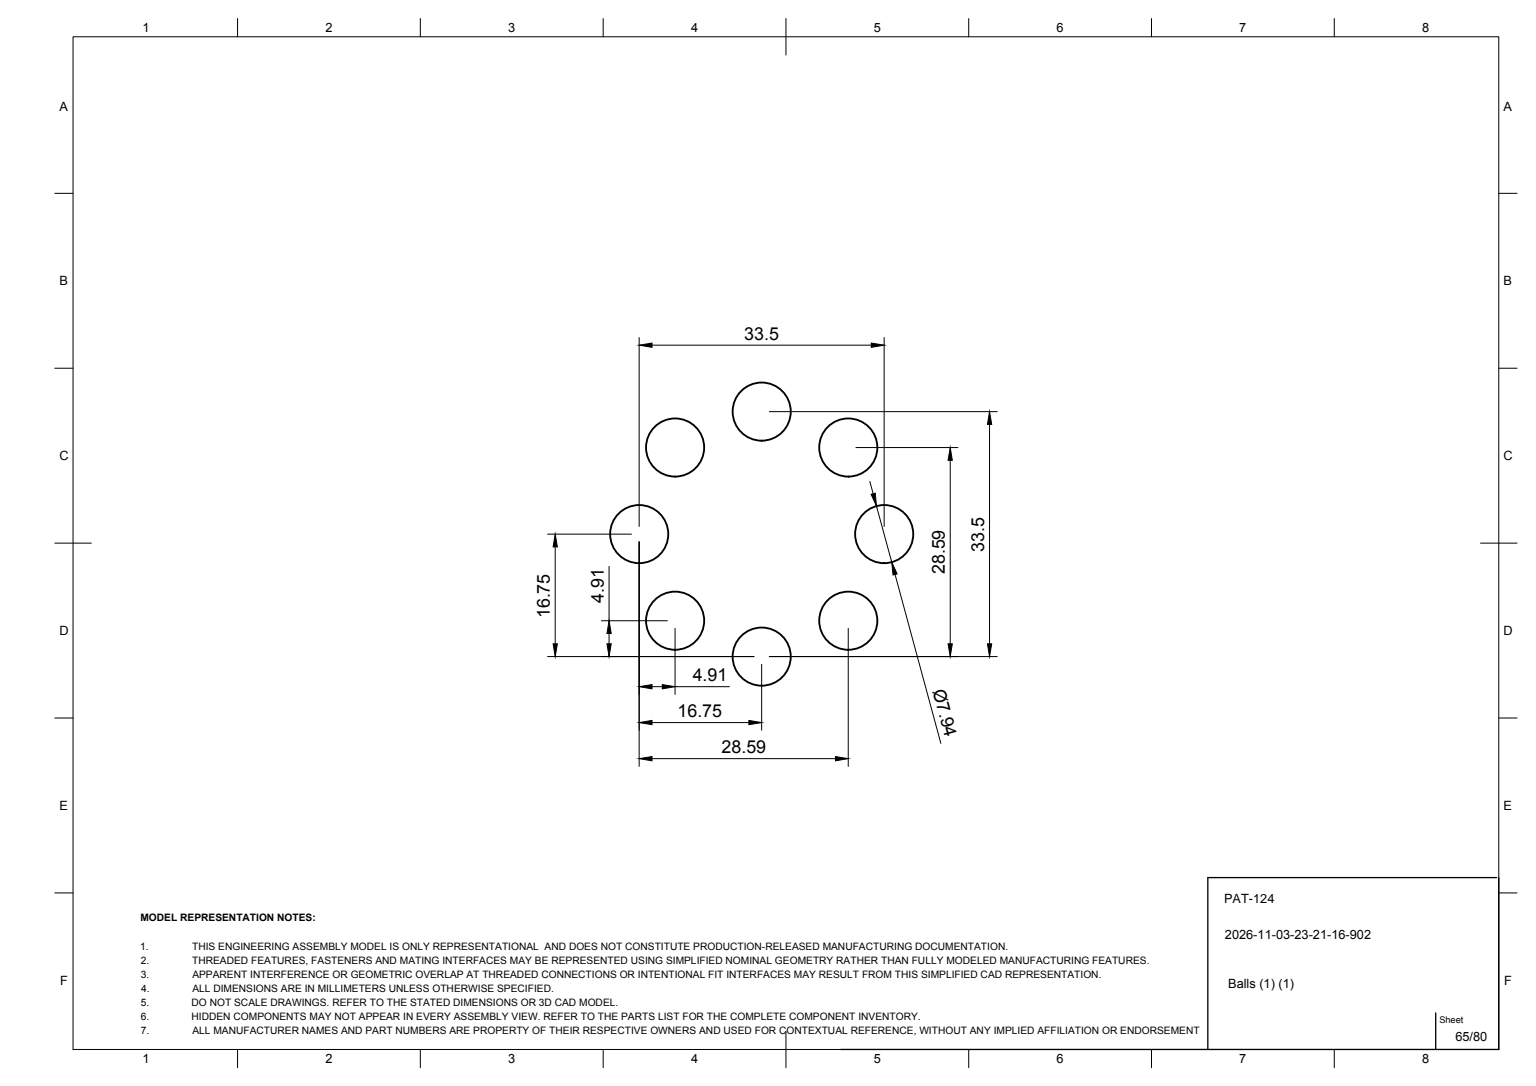
ISO-10303-21;
HEADER;
/* Generated by software containing ST-Developer
 * from STEP Tools, Inc. (www.steptools.com) 
 */

FILE_DESCRIPTION(
/* description */ ('XY cross-slide table'),
/* implementation_level */ '2;1');

FILE_NAME(
/* name */ 'Balls (1) (1).step',
/* time_stamp */ '2026-10-28T03:22:46-07:00',
/* author */ (''),
/* organization */ (''),
/* preprocessor_version */ 'ST-DEVELOPER v20.2',
/* originating_system */ 'Autodesk Translation Framework v15.17.0.0',
/* authorisation */ '');

FILE_SCHEMA (('AUTOMOTIVE_DESIGN { 1 0 10303 214 3 1 1 }'));
ENDSEC;

DATA;
#10=MECHANICAL_DESIGN_GEOMETRIC_PRESENTATION_REPRESENTATION('',(#1750,#1751,#1752,#1753,#1754,#1755,#1756,#1757),#62984);
#1425=SPHERICAL_SURFACE('',#25700,0.3969);
#1426=SPHERICAL_SURFACE('',#25702,0.3969);
#1427=SPHERICAL_SURFACE('',#25704,0.3969);
#1428=SPHERICAL_SURFACE('',#25706,0.3969);
#1429=SPHERICAL_SURFACE('',#25708,0.3969);
#1430=SPHERICAL_SURFACE('',#25710,0.3969);
#1431=SPHERICAL_SURFACE('',#25712,0.3969);
#1432=SPHERICAL_SURFACE('',#25714,0.3969);
#1562=SHAPE_REPRESENTATION_RELATIONSHIP('SRR','None',#63419,#1645);
#1645=ADVANCED_BREP_SHAPE_REPRESENTATION('',(#1859,#1860,#1861,#1862,#1863,
#1864,#1865,#1866),#62956);
#1750=STYLED_ITEM('',(#63905),#1859);
#1751=STYLED_ITEM('',(#63905),#1860);
#1752=STYLED_ITEM('',(#63905),#1861);
#1753=STYLED_ITEM('',(#63905),#1862);
#1754=STYLED_ITEM('',(#63905),#1863);
#1755=STYLED_ITEM('',(#63905),#1864);
#1756=STYLED_ITEM('',(#63905),#1865);
#1757=STYLED_ITEM('',(#63905),#1866);
#1859=MANIFOLD_SOLID_BREP('Body1',#23048);
#1860=MANIFOLD_SOLID_BREP('Body2',#23049);
#1861=MANIFOLD_SOLID_BREP('Body3',#23050);
#1862=MANIFOLD_SOLID_BREP('Body4',#23051);
#1863=MANIFOLD_SOLID_BREP('Body5',#23052);
#1864=MANIFOLD_SOLID_BREP('Body6',#23053);
#1865=MANIFOLD_SOLID_BREP('Body7',#23054);
#1866=MANIFOLD_SOLID_BREP('Body8',#23055);
#3739=FACE_OUTER_BOUND('',#5380,.T.);
#3740=FACE_OUTER_BOUND('',#5381,.T.);
#3741=FACE_OUTER_BOUND('',#5382,.T.);
#3742=FACE_OUTER_BOUND('',#5383,.T.);
#3743=FACE_OUTER_BOUND('',#5384,.T.);
#3744=FACE_OUTER_BOUND('',#5385,.T.);
#3745=FACE_OUTER_BOUND('',#5386,.T.);
#3746=FACE_OUTER_BOUND('',#5387,.T.);
#5380=EDGE_LOOP('',(#18890,#18891));
#5381=EDGE_LOOP('',(#18892,#18893));
#5382=EDGE_LOOP('',(#18894,#18895));
#5383=EDGE_LOOP('',(#18896,#18897));
#5384=EDGE_LOOP('',(#18898,#18899));
#5385=EDGE_LOOP('',(#18900,#18901));
#5386=EDGE_LOOP('',(#18902,#18903));
#5387=EDGE_LOOP('',(#18904,#18905));
#9558=CIRCLE('',#25701,0.3969);
#9559=CIRCLE('',#25703,0.3969);
#9560=CIRCLE('',#25705,0.3969);
#9561=CIRCLE('',#25707,0.3969);
#9562=CIRCLE('',#25709,0.3969);
#9563=CIRCLE('',#25711,0.3969);
#9564=CIRCLE('',#25713,0.3969);
#9565=CIRCLE('',#25715,0.3969);
#11115=VERTEX_POINT('',#49131);
#11116=VERTEX_POINT('',#49132);
#11117=VERTEX_POINT('',#49135);
#11118=VERTEX_POINT('',#49136);
#11119=VERTEX_POINT('',#49139);
#11120=VERTEX_POINT('',#49140);
#11121=VERTEX_POINT('',#49143);
#11122=VERTEX_POINT('',#49144);
#11123=VERTEX_POINT('',#49147);
#11124=VERTEX_POINT('',#49148);
#11125=VERTEX_POINT('',#49151);
#11126=VERTEX_POINT('',#49152);
#11127=VERTEX_POINT('',#49155);
#11128=VERTEX_POINT('',#49156);
#11129=VERTEX_POINT('',#49159);
#11130=VERTEX_POINT('',#49160);
#13829=EDGE_CURVE('',#11115,#11116,#9558,.T.);
#13830=EDGE_CURVE('',#11117,#11118,#9559,.T.);
#13831=EDGE_CURVE('',#11119,#11120,#9560,.T.);
#13832=EDGE_CURVE('',#11121,#11122,#9561,.T.);
#13833=EDGE_CURVE('',#11123,#11124,#9562,.T.);
#13834=EDGE_CURVE('',#11125,#11126,#9563,.T.);
#13835=EDGE_CURVE('',#11127,#11128,#9564,.T.);
#13836=EDGE_CURVE('',#11129,#11130,#9565,.T.);
#18890=ORIENTED_EDGE('',*,*,#13829,.T.);
#18891=ORIENTED_EDGE('',*,*,#13829,.F.);
#18892=ORIENTED_EDGE('',*,*,#13830,.T.);
#18893=ORIENTED_EDGE('',*,*,#13830,.F.);
#18894=ORIENTED_EDGE('',*,*,#13831,.T.);
#18895=ORIENTED_EDGE('',*,*,#13831,.F.);
#18896=ORIENTED_EDGE('',*,*,#13832,.T.);
#18897=ORIENTED_EDGE('',*,*,#13832,.F.);
#18898=ORIENTED_EDGE('',*,*,#13833,.T.);
#18899=ORIENTED_EDGE('',*,*,#13833,.F.);
#18900=ORIENTED_EDGE('',*,*,#13834,.T.);
#18901=ORIENTED_EDGE('',*,*,#13834,.F.);
#18902=ORIENTED_EDGE('',*,*,#13835,.T.);
#18903=ORIENTED_EDGE('',*,*,#13835,.F.);
#18904=ORIENTED_EDGE('',*,*,#13836,.T.);
#18905=ORIENTED_EDGE('',*,*,#13836,.F.);
#22520=ADVANCED_FACE('',(#3739),#1425,.T.);
#22521=ADVANCED_FACE('',(#3740),#1426,.T.);
#22522=ADVANCED_FACE('',(#3741),#1427,.T.);
#22523=ADVANCED_FACE('',(#3742),#1428,.T.);
#22524=ADVANCED_FACE('',(#3743),#1429,.T.);
#22525=ADVANCED_FACE('',(#3744),#1430,.T.);
#22526=ADVANCED_FACE('',(#3745),#1431,.T.);
#22527=ADVANCED_FACE('',(#3746),#1432,.T.);
#23048=CLOSED_SHELL('',(#22520));
#23049=CLOSED_SHELL('',(#22521));
#23050=CLOSED_SHELL('',(#22522));
#23051=CLOSED_SHELL('',(#22523));
#23052=CLOSED_SHELL('',(#22524));
#23053=CLOSED_SHELL('',(#22525));
#23054=CLOSED_SHELL('',(#22526));
#23055=CLOSED_SHELL('',(#22527));
#25699=AXIS2_PLACEMENT_3D('',#49129,#30816,#30817);
#25700=AXIS2_PLACEMENT_3D('',#49130,#30818,#30819);
#25701=AXIS2_PLACEMENT_3D('',#49133,#30820,#30821);
#25702=AXIS2_PLACEMENT_3D('',#49134,#30822,#30823);
#25703=AXIS2_PLACEMENT_3D('',#49137,#30824,#30825);
#25704=AXIS2_PLACEMENT_3D('',#49138,#30826,#30827);
#25705=AXIS2_PLACEMENT_3D('',#49141,#30828,#30829);
#25706=AXIS2_PLACEMENT_3D('',#49142,#30830,#30831);
#25707=AXIS2_PLACEMENT_3D('',#49145,#30832,#30833);
#25708=AXIS2_PLACEMENT_3D('',#49146,#30834,#30835);
#25709=AXIS2_PLACEMENT_3D('',#49149,#30836,#30837);
#25710=AXIS2_PLACEMENT_3D('',#49150,#30838,#30839);
#25711=AXIS2_PLACEMENT_3D('',#49153,#30840,#30841);
#25712=AXIS2_PLACEMENT_3D('',#49154,#30842,#30843);
#25713=AXIS2_PLACEMENT_3D('',#49157,#30844,#30845);
#25714=AXIS2_PLACEMENT_3D('',#49158,#30846,#30847);
#25715=AXIS2_PLACEMENT_3D('',#49161,#30848,#30849);
#30816=DIRECTION('axis',(0.,0.,1.));
#30817=DIRECTION('refdir',(1.,0.,0.));
#30818=DIRECTION('center_axis',(0.,0.,1.));
#30819=DIRECTION('ref_axis',(1.,0.,0.));
#30820=DIRECTION('center_axis',(1.22464679914735E-16,-1.,0.));
#30821=DIRECTION('ref_axis',(-1.,-1.22464679914735E-16,0.));
#30822=DIRECTION('center_axis',(0.707106781186548,0.,0.707106781186548));
#30823=DIRECTION('ref_axis',(0.707106781186548,0.,-0.707106781186548));
#30824=DIRECTION('center_axis',(8.65956056235493E-17,-1.,-8.65956056235493E-17));
#30825=DIRECTION('ref_axis',(-0.707106781186548,-1.22464679914735E-16,0.707106781186548));
#30826=DIRECTION('center_axis',(1.,0.,0.));
#30827=DIRECTION('ref_axis',(6.12323399573677E-17,0.,-1.));
#30828=DIRECTION('center_axis',(7.49879891330929E-33,-1.,-1.22464679914735E-16));
#30829=DIRECTION('ref_axis',(-6.12323399573677E-17,-1.22464679914735E-16,
1.));
#30830=DIRECTION('center_axis',(0.707106781186548,0.,-0.707106781186548));
#30831=DIRECTION('ref_axis',(-0.707106781186548,0.,-0.707106781186548));
#30832=DIRECTION('center_axis',(-8.65956056235493E-17,-1.,-8.65956056235493E-17));
#30833=DIRECTION('ref_axis',(0.707106781186548,-1.22464679914735E-16,0.707106781186548));
#30834=DIRECTION('center_axis',(0.,0.,-1.));
#30835=DIRECTION('ref_axis',(-1.,0.,-1.22464679914735E-16));
#30836=DIRECTION('center_axis',(-1.22464679914735E-16,-1.,-1.49975978266186E-32));
#30837=DIRECTION('ref_axis',(1.,-1.22464679914735E-16,1.22464679914735E-16));
#30838=DIRECTION('center_axis',(-0.707106781186548,0.,-0.707106781186548));
#30839=DIRECTION('ref_axis',(-0.707106781186548,0.,0.707106781186548));
#30840=DIRECTION('center_axis',(-8.65956056235493E-17,-1.,8.65956056235493E-17));
#30841=DIRECTION('ref_axis',(0.707106781186548,-1.22464679914735E-16,-0.707106781186548));
#30842=DIRECTION('center_axis',(-1.,0.,0.));
#30843=DIRECTION('ref_axis',(-1.83697019872103E-16,0.,1.));
#30844=DIRECTION('center_axis',(-2.24963967399279E-32,-1.,1.22464679914735E-16));
#30845=DIRECTION('ref_axis',(1.83697019872103E-16,-1.22464679914735E-16,
-1.));
#30846=DIRECTION('center_axis',(-0.707106781186548,0.,0.707106781186548));
#30847=DIRECTION('ref_axis',(0.707106781186548,0.,0.707106781186548));
#30848=DIRECTION('center_axis',(8.65956056235493E-17,-1.,8.65956056235494E-17));
#30849=DIRECTION('ref_axis',(-0.707106781186548,-1.22464679914735E-16,-0.707106781186548));
#49129=CARTESIAN_POINT('',(0.,0.,0.));
#49130=CARTESIAN_POINT('Origin',(1.675,0.,0.));
#49131=CARTESIAN_POINT('',(1.675,-2.97627328869245E-33,0.3969));
#49132=CARTESIAN_POINT('',(1.675,-2.97627328869245E-33,-0.3969));
#49133=CARTESIAN_POINT('Origin',(1.675,0.,0.));
#49134=CARTESIAN_POINT('Origin',(1.18440385848747,0.,-1.18440385848747));
#49135=CARTESIAN_POINT('',(1.46505453994041,3.1867025333467E-33,-0.903753177034526));
#49136=CARTESIAN_POINT('',(0.903753177034527,-9.13924911073161E-33,-1.46505453994041));
#49137=CARTESIAN_POINT('Origin',(1.18440385848747,0.,-1.18440385848747));
#49138=CARTESIAN_POINT('Origin',(1.02564169428591E-16,0.,-1.675));
#49139=CARTESIAN_POINT('',(0.3969,-2.97627328869246E-33,-1.675));
#49140=CARTESIAN_POINT('',(-0.3969,-2.97627328869245E-33,-1.675));
#49141=CARTESIAN_POINT('Origin',(1.02564169428591E-16,0.,-1.675));
#49142=CARTESIAN_POINT('Origin',(-1.18440385848747,0.,-1.18440385848747));
#49143=CARTESIAN_POINT('',(-0.903753177034526,3.1867025333467E-33,-1.46505453994041));
#49144=CARTESIAN_POINT('',(-1.46505453994041,-9.13924911073161E-33,-0.903753177034527));
#49145=CARTESIAN_POINT('Origin',(-1.18440385848747,0.,-1.18440385848747));
#49146=CARTESIAN_POINT('Origin',(-1.675,0.,-2.05128338857182E-16));
#49147=CARTESIAN_POINT('',(-1.675,-2.97627328869246E-33,-0.3969));
#49148=CARTESIAN_POINT('',(-1.675,-2.97627328869245E-33,0.3969));
#49149=CARTESIAN_POINT('Origin',(-1.675,0.,-2.05128338857182E-16));
#49150=CARTESIAN_POINT('Origin',(-1.18440385848747,0.,1.18440385848747));
#49151=CARTESIAN_POINT('',(-1.46505453994041,6.26819044436628E-33,0.903753177034526));
#49152=CARTESIAN_POINT('',(-0.903753177034527,-1.22207370217512E-32,1.46505453994041));
#49153=CARTESIAN_POINT('Origin',(-1.18440385848747,0.,1.18440385848747));
#49154=CARTESIAN_POINT('Origin',(-3.07692508285772E-16,0.,1.675));
#49155=CARTESIAN_POINT('',(-0.3969,-2.97627328869246E-33,1.675));
#49156=CARTESIAN_POINT('',(0.396899999999999,-2.97627328869245E-33,1.675));
#49157=CARTESIAN_POINT('Origin',(-3.07692508285772E-16,0.,1.675));
#49158=CARTESIAN_POINT('Origin',(1.18440385848747,0.,1.18440385848747));
#49159=CARTESIAN_POINT('',(0.903753177034526,9.34967835538585E-33,1.46505453994041));
#49160=CARTESIAN_POINT('',(1.46505453994041,-1.53022249327708E-32,0.903753177034527));
#49161=CARTESIAN_POINT('Origin',(1.18440385848747,0.,1.18440385848747));
#62857=UNCERTAINTY_MEASURE_WITH_UNIT(LENGTH_MEASURE(0.001),#62985,
'DISTANCE_ACCURACY_VALUE',
'Maximum model space distance between geometric entities at asserted c
onnectivities');
#62885=UNCERTAINTY_MEASURE_WITH_UNIT(LENGTH_MEASURE(0.001),#62985,
'DISTANCE_ACCURACY_VALUE',
'Maximum model space distance between geometric entities at asserted c
onnectivities');
#62956=(
GEOMETRIC_REPRESENTATION_CONTEXT(3)
GLOBAL_UNCERTAINTY_ASSIGNED_CONTEXT((#62857))
GLOBAL_UNIT_ASSIGNED_CONTEXT((#62985,#62987,#62988))
REPRESENTATION_CONTEXT('','3D')
);
#62984=(
GEOMETRIC_REPRESENTATION_CONTEXT(3)
GLOBAL_UNCERTAINTY_ASSIGNED_CONTEXT((#62885))
GLOBAL_UNIT_ASSIGNED_CONTEXT((#62985,#62987,#62988))
REPRESENTATION_CONTEXT('','3D')
);
#62985=(
LENGTH_UNIT()
NAMED_UNIT(*)
SI_UNIT(.CENTI.,.METRE.)
);
#62987=(
NAMED_UNIT(*)
PLANE_ANGLE_UNIT()
SI_UNIT($,.RADIAN.)
);
#62988=(
NAMED_UNIT(*)
SI_UNIT($,.STERADIAN.)
SOLID_ANGLE_UNIT()
);
#63059=SHAPE_DEFINITION_REPRESENTATION(#63242,#63419);
#63242=PRODUCT_DEFINITION_SHAPE('',$,#63518);
#63419=SHAPE_REPRESENTATION('',(#25699),#62956);
#63447=PRODUCT_DEFINITION_CONTEXT('part definition',#63743,'design');
#63518=PRODUCT_DEFINITION('Balls (1) (1)','Balls (1) (1)',#63616,#63447);
#63616=PRODUCT_DEFINITION_FORMATION('',$,#63815);
#63743=APPLICATION_CONTEXT(
'Core Data for Automotive Mechanical Design Process');
#63744=PRODUCT_CONTEXT('part definition',#63743,'mechanical');
#63815=PRODUCT('Balls (1) (1)','Balls (1) (1)','Balls (1) (1)',(#63744));
#63899=COLOUR_RGB('Sky Blue',0.24,0.69,0.87);
#63900=FILL_AREA_STYLE_COLOUR('',#63899);
#63901=FILL_AREA_STYLE('',(#63900));
#63902=SURFACE_STYLE_FILL_AREA(#63901);
#63903=SURFACE_SIDE_STYLE('',(#63902));
#63904=SURFACE_STYLE_USAGE(.BOTH.,#63903);
#63905=PRESENTATION_STYLE_ASSIGNMENT((#63904));
ENDSEC;
END-ISO-10303-21;
